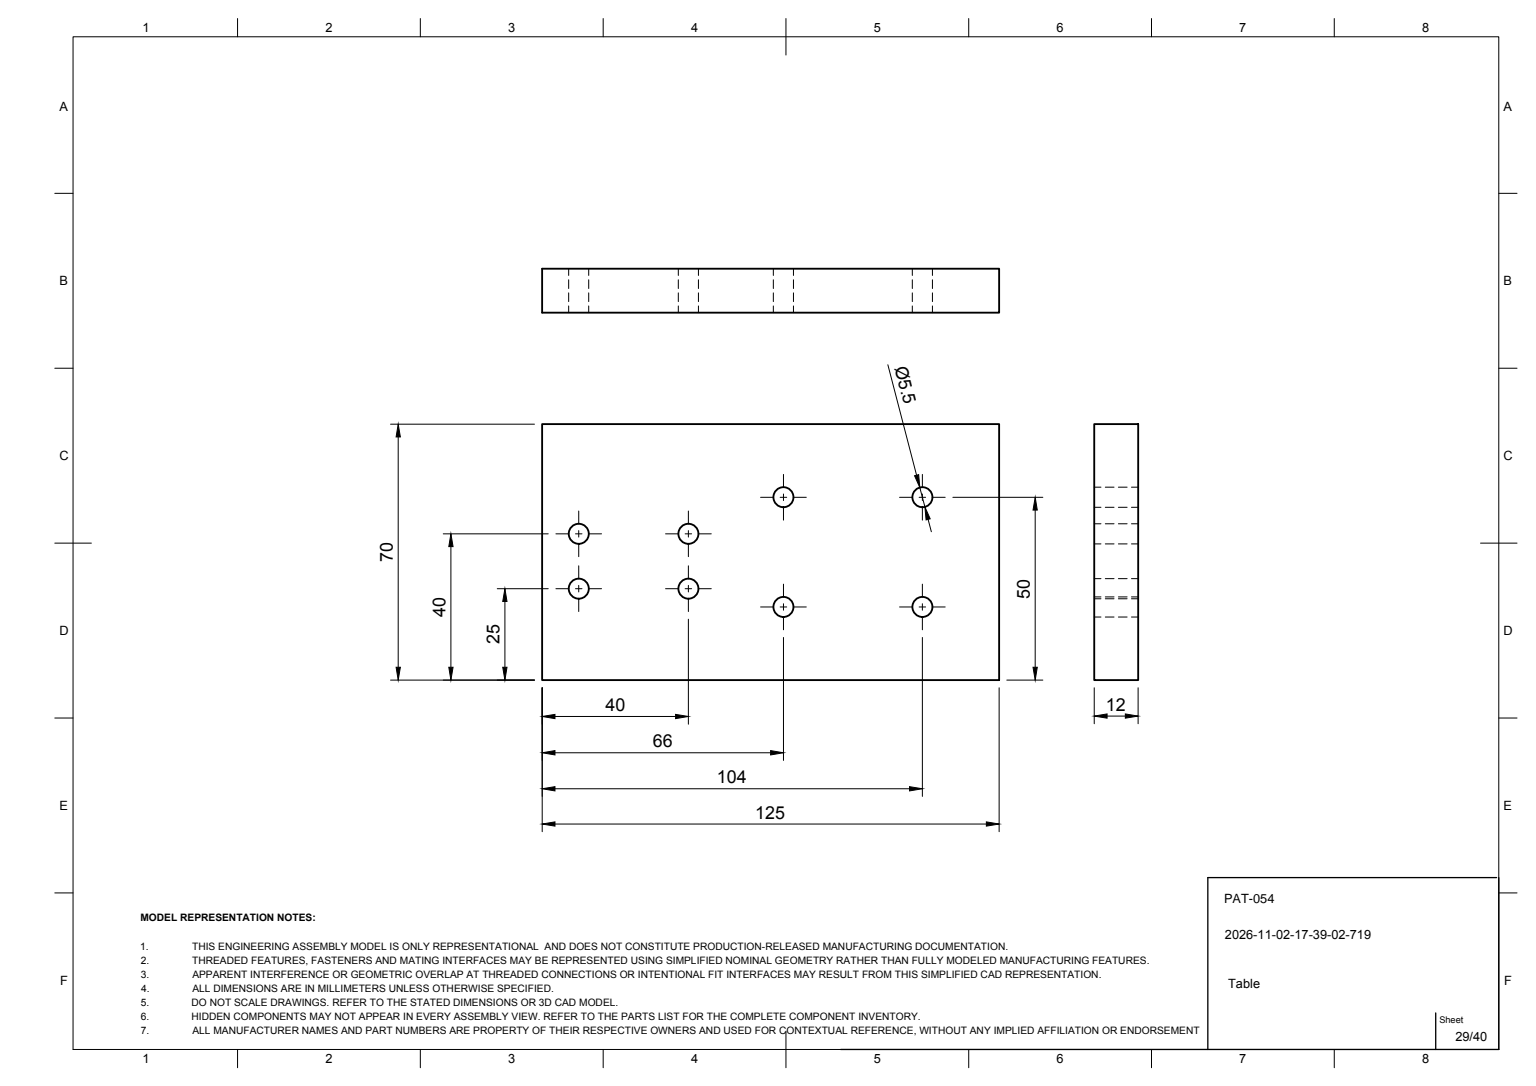
ISO-10303-21;
HEADER;
/* Generated by software containing ST-Developer
 * from STEP Tools, Inc. (www.steptools.com) 
 */

FILE_DESCRIPTION(
/* description */ ('PAT-054'),
/* implementation_level */ '2;1');

FILE_NAME(
/* name */ 'Table.step',
/* time_stamp */ '2026-10-29T16:38:13-07:00',
/* author */ (''),
/* organization */ (''),
/* preprocessor_version */ 'ST-DEVELOPER v20.2',
/* originating_system */ 'Autodesk Translation Framework v15.17.0.0',
/* authorisation */ '');

FILE_SCHEMA (('AUTOMOTIVE_DESIGN { 1 0 10303 214 3 1 1 }'));
ENDSEC;

DATA;
#10=MECHANICAL_DESIGN_GEOMETRIC_PRESENTATION_REPRESENTATION('',(#938),#33981);
#835=SHAPE_REPRESENTATION_RELATIONSHIP('SRR','None',#34211,#879);
#879=ADVANCED_BREP_SHAPE_REPRESENTATION('',(#996),#33959);
#938=STYLED_ITEM('',(#34531),#996);
#996=MANIFOLD_SOLID_BREP('Body1',#13050);
#1160=FACE_BOUND('',#2799,.T.);
#1161=FACE_BOUND('',#2800,.T.);
#1162=FACE_BOUND('',#2801,.T.);
#1163=FACE_BOUND('',#2802,.T.);
#1164=FACE_BOUND('',#2803,.T.);
#1165=FACE_BOUND('',#2804,.T.);
#1166=FACE_BOUND('',#2805,.T.);
#1167=FACE_BOUND('',#2806,.T.);
#1168=FACE_BOUND('',#2808,.T.);
#1169=FACE_BOUND('',#2809,.T.);
#1170=FACE_BOUND('',#2810,.T.);
#1171=FACE_BOUND('',#2811,.T.);
#1172=FACE_BOUND('',#2812,.T.);
#1173=FACE_BOUND('',#2813,.T.);
#1174=FACE_BOUND('',#2814,.T.);
#1175=FACE_BOUND('',#2815,.T.);
#1418=PLANE('',#14280);
#1419=PLANE('',#14281);
#1420=PLANE('',#14282);
#1421=PLANE('',#14283);
#1422=PLANE('',#14284);
#1423=PLANE('',#14285);
#1915=FACE_OUTER_BOUND('',#2786,.T.);
#1916=FACE_OUTER_BOUND('',#2787,.T.);
#1917=FACE_OUTER_BOUND('',#2788,.T.);
#1918=FACE_OUTER_BOUND('',#2789,.T.);
#1919=FACE_OUTER_BOUND('',#2790,.T.);
#1920=FACE_OUTER_BOUND('',#2791,.T.);
#1921=FACE_OUTER_BOUND('',#2792,.T.);
#1922=FACE_OUTER_BOUND('',#2793,.T.);
#1923=FACE_OUTER_BOUND('',#2794,.T.);
#1924=FACE_OUTER_BOUND('',#2795,.T.);
#1925=FACE_OUTER_BOUND('',#2796,.T.);
#1926=FACE_OUTER_BOUND('',#2797,.T.);
#1927=FACE_OUTER_BOUND('',#2798,.T.);
#1928=FACE_OUTER_BOUND('',#2807,.T.);
#2786=EDGE_LOOP('',(#10085,#10086,#10087,#10088));
#2787=EDGE_LOOP('',(#10089,#10090,#10091,#10092));
#2788=EDGE_LOOP('',(#10093,#10094,#10095,#10096));
#2789=EDGE_LOOP('',(#10097,#10098,#10099,#10100));
#2790=EDGE_LOOP('',(#10101,#10102,#10103,#10104));
#2791=EDGE_LOOP('',(#10105,#10106,#10107,#10108));
#2792=EDGE_LOOP('',(#10109,#10110,#10111,#10112));
#2793=EDGE_LOOP('',(#10113,#10114,#10115,#10116));
#2794=EDGE_LOOP('',(#10117,#10118,#10119,#10120));
#2795=EDGE_LOOP('',(#10121,#10122,#10123,#10124));
#2796=EDGE_LOOP('',(#10125,#10126,#10127,#10128));
#2797=EDGE_LOOP('',(#10129,#10130,#10131,#10132));
#2798=EDGE_LOOP('',(#10133,#10134,#10135,#10136));
#2799=EDGE_LOOP('',(#10137));
#2800=EDGE_LOOP('',(#10138));
#2801=EDGE_LOOP('',(#10139));
#2802=EDGE_LOOP('',(#10140));
#2803=EDGE_LOOP('',(#10141));
#2804=EDGE_LOOP('',(#10142));
#2805=EDGE_LOOP('',(#10143));
#2806=EDGE_LOOP('',(#10144));
#2807=EDGE_LOOP('',(#10145,#10146,#10147,#10148));
#2808=EDGE_LOOP('',(#10149));
#2809=EDGE_LOOP('',(#10150));
#2810=EDGE_LOOP('',(#10151));
#2811=EDGE_LOOP('',(#10152));
#2812=EDGE_LOOP('',(#10153));
#2813=EDGE_LOOP('',(#10154));
#2814=EDGE_LOOP('',(#10155));
#2815=EDGE_LOOP('',(#10156));
#3686=LINE('',#20848,#4620);
#3687=LINE('',#20854,#4621);
#3688=LINE('',#20860,#4622);
#3689=LINE('',#20866,#4623);
#3690=LINE('',#20872,#4624);
#3691=LINE('',#20878,#4625);
#3692=LINE('',#20884,#4626);
#3693=LINE('',#20890,#4627);
#3694=LINE('',#20895,#4628);
#3695=LINE('',#20897,#4629);
#3696=LINE('',#20899,#4630);
#3697=LINE('',#20900,#4631);
#3698=LINE('',#20903,#4632);
#3699=LINE('',#20905,#4633);
#3700=LINE('',#20906,#4634);
#3701=LINE('',#20909,#4635);
#3702=LINE('',#20911,#4636);
#3703=LINE('',#20912,#4637);
#3704=LINE('',#20914,#4638);
#3705=LINE('',#20915,#4639);
#4620=VECTOR('',#16737,0.275);
#4621=VECTOR('',#16744,0.275);
#4622=VECTOR('',#16751,0.275);
#4623=VECTOR('',#16758,0.275);
#4624=VECTOR('',#16765,0.275);
#4625=VECTOR('',#16772,0.275);
#4626=VECTOR('',#16779,0.275);
#4627=VECTOR('',#16786,0.275);
#4628=VECTOR('',#16791,1.);
#4629=VECTOR('',#16792,1.);
#4630=VECTOR('',#16793,1.);
#4631=VECTOR('',#16794,1.);
#4632=VECTOR('',#16797,1.);
#4633=VECTOR('',#16798,1.);
#4634=VECTOR('',#16799,1.);
#4635=VECTOR('',#16802,1.);
#4636=VECTOR('',#16803,1.);
#4637=VECTOR('',#16804,1.);
#4638=VECTOR('',#16807,1.);
#4639=VECTOR('',#16808,1.);
#5420=CIRCLE('',#14257,0.275);
#5421=CIRCLE('',#14258,0.275);
#5422=CIRCLE('',#14260,0.275);
#5423=CIRCLE('',#14261,0.275);
#5424=CIRCLE('',#14263,0.275);
#5425=CIRCLE('',#14264,0.275);
#5426=CIRCLE('',#14266,0.275);
#5427=CIRCLE('',#14267,0.275);
#5428=CIRCLE('',#14269,0.275);
#5429=CIRCLE('',#14270,0.275);
#5430=CIRCLE('',#14272,0.275);
#5431=CIRCLE('',#14273,0.275);
#5432=CIRCLE('',#14275,0.275);
#5433=CIRCLE('',#14276,0.275);
#5434=CIRCLE('',#14278,0.275);
#5435=CIRCLE('',#14279,0.275);
#6118=VERTEX_POINT('',#20845);
#6119=VERTEX_POINT('',#20847);
#6120=VERTEX_POINT('',#20851);
#6121=VERTEX_POINT('',#20853);
#6122=VERTEX_POINT('',#20857);
#6123=VERTEX_POINT('',#20859);
#6124=VERTEX_POINT('',#20863);
#6125=VERTEX_POINT('',#20865);
#6126=VERTEX_POINT('',#20869);
#6127=VERTEX_POINT('',#20871);
#6128=VERTEX_POINT('',#20875);
#6129=VERTEX_POINT('',#20877);
#6130=VERTEX_POINT('',#20881);
#6131=VERTEX_POINT('',#20883);
#6132=VERTEX_POINT('',#20887);
#6133=VERTEX_POINT('',#20889);
#6134=VERTEX_POINT('',#20893);
#6135=VERTEX_POINT('',#20894);
#6136=VERTEX_POINT('',#20896);
#6137=VERTEX_POINT('',#20898);
#6138=VERTEX_POINT('',#20902);
#6139=VERTEX_POINT('',#20904);
#6140=VERTEX_POINT('',#20908);
#6141=VERTEX_POINT('',#20910);
#7542=EDGE_CURVE('',#6118,#6118,#5420,.T.);
#7543=EDGE_CURVE('',#6118,#6119,#3686,.T.);
#7544=EDGE_CURVE('',#6119,#6119,#5421,.T.);
#7545=EDGE_CURVE('',#6120,#6120,#5422,.T.);
#7546=EDGE_CURVE('',#6120,#6121,#3687,.T.);
#7547=EDGE_CURVE('',#6121,#6121,#5423,.T.);
#7548=EDGE_CURVE('',#6122,#6122,#5424,.T.);
#7549=EDGE_CURVE('',#6122,#6123,#3688,.T.);
#7550=EDGE_CURVE('',#6123,#6123,#5425,.T.);
#7551=EDGE_CURVE('',#6124,#6124,#5426,.T.);
#7552=EDGE_CURVE('',#6124,#6125,#3689,.T.);
#7553=EDGE_CURVE('',#6125,#6125,#5427,.T.);
#7554=EDGE_CURVE('',#6126,#6126,#5428,.T.);
#7555=EDGE_CURVE('',#6126,#6127,#3690,.T.);
#7556=EDGE_CURVE('',#6127,#6127,#5429,.T.);
#7557=EDGE_CURVE('',#6128,#6128,#5430,.T.);
#7558=EDGE_CURVE('',#6128,#6129,#3691,.T.);
#7559=EDGE_CURVE('',#6129,#6129,#5431,.T.);
#7560=EDGE_CURVE('',#6130,#6130,#5432,.T.);
#7561=EDGE_CURVE('',#6130,#6131,#3692,.T.);
#7562=EDGE_CURVE('',#6131,#6131,#5433,.T.);
#7563=EDGE_CURVE('',#6132,#6132,#5434,.T.);
#7564=EDGE_CURVE('',#6132,#6133,#3693,.T.);
#7565=EDGE_CURVE('',#6133,#6133,#5435,.T.);
#7566=EDGE_CURVE('',#6134,#6135,#3694,.T.);
#7567=EDGE_CURVE('',#6135,#6136,#3695,.T.);
#7568=EDGE_CURVE('',#6137,#6136,#3696,.T.);
#7569=EDGE_CURVE('',#6134,#6137,#3697,.T.);
#7570=EDGE_CURVE('',#6138,#6134,#3698,.T.);
#7571=EDGE_CURVE('',#6139,#6137,#3699,.T.);
#7572=EDGE_CURVE('',#6138,#6139,#3700,.T.);
#7573=EDGE_CURVE('',#6140,#6138,#3701,.T.);
#7574=EDGE_CURVE('',#6141,#6139,#3702,.T.);
#7575=EDGE_CURVE('',#6140,#6141,#3703,.T.);
#7576=EDGE_CURVE('',#6135,#6140,#3704,.T.);
#7577=EDGE_CURVE('',#6136,#6141,#3705,.T.);
#10085=ORIENTED_EDGE('',*,*,#7542,.F.);
#10086=ORIENTED_EDGE('',*,*,#7543,.T.);
#10087=ORIENTED_EDGE('',*,*,#7544,.F.);
#10088=ORIENTED_EDGE('',*,*,#7543,.F.);
#10089=ORIENTED_EDGE('',*,*,#7545,.F.);
#10090=ORIENTED_EDGE('',*,*,#7546,.T.);
#10091=ORIENTED_EDGE('',*,*,#7547,.F.);
#10092=ORIENTED_EDGE('',*,*,#7546,.F.);
#10093=ORIENTED_EDGE('',*,*,#7548,.F.);
#10094=ORIENTED_EDGE('',*,*,#7549,.T.);
#10095=ORIENTED_EDGE('',*,*,#7550,.F.);
#10096=ORIENTED_EDGE('',*,*,#7549,.F.);
#10097=ORIENTED_EDGE('',*,*,#7551,.F.);
#10098=ORIENTED_EDGE('',*,*,#7552,.T.);
#10099=ORIENTED_EDGE('',*,*,#7553,.F.);
#10100=ORIENTED_EDGE('',*,*,#7552,.F.);
#10101=ORIENTED_EDGE('',*,*,#7554,.F.);
#10102=ORIENTED_EDGE('',*,*,#7555,.T.);
#10103=ORIENTED_EDGE('',*,*,#7556,.F.);
#10104=ORIENTED_EDGE('',*,*,#7555,.F.);
#10105=ORIENTED_EDGE('',*,*,#7557,.F.);
#10106=ORIENTED_EDGE('',*,*,#7558,.T.);
#10107=ORIENTED_EDGE('',*,*,#7559,.F.);
#10108=ORIENTED_EDGE('',*,*,#7558,.F.);
#10109=ORIENTED_EDGE('',*,*,#7560,.F.);
#10110=ORIENTED_EDGE('',*,*,#7561,.T.);
#10111=ORIENTED_EDGE('',*,*,#7562,.F.);
#10112=ORIENTED_EDGE('',*,*,#7561,.F.);
#10113=ORIENTED_EDGE('',*,*,#7563,.F.);
#10114=ORIENTED_EDGE('',*,*,#7564,.T.);
#10115=ORIENTED_EDGE('',*,*,#7565,.F.);
#10116=ORIENTED_EDGE('',*,*,#7564,.F.);
#10117=ORIENTED_EDGE('',*,*,#7566,.T.);
#10118=ORIENTED_EDGE('',*,*,#7567,.T.);
#10119=ORIENTED_EDGE('',*,*,#7568,.F.);
#10120=ORIENTED_EDGE('',*,*,#7569,.F.);
#10121=ORIENTED_EDGE('',*,*,#7570,.T.);
#10122=ORIENTED_EDGE('',*,*,#7569,.T.);
#10123=ORIENTED_EDGE('',*,*,#7571,.F.);
#10124=ORIENTED_EDGE('',*,*,#7572,.F.);
#10125=ORIENTED_EDGE('',*,*,#7573,.T.);
#10126=ORIENTED_EDGE('',*,*,#7572,.T.);
#10127=ORIENTED_EDGE('',*,*,#7574,.F.);
#10128=ORIENTED_EDGE('',*,*,#7575,.F.);
#10129=ORIENTED_EDGE('',*,*,#7576,.T.);
#10130=ORIENTED_EDGE('',*,*,#7575,.T.);
#10131=ORIENTED_EDGE('',*,*,#7577,.F.);
#10132=ORIENTED_EDGE('',*,*,#7567,.F.);
#10133=ORIENTED_EDGE('',*,*,#7577,.T.);
#10134=ORIENTED_EDGE('',*,*,#7574,.T.);
#10135=ORIENTED_EDGE('',*,*,#7571,.T.);
#10136=ORIENTED_EDGE('',*,*,#7568,.T.);
#10137=ORIENTED_EDGE('',*,*,#7565,.T.);
#10138=ORIENTED_EDGE('',*,*,#7562,.T.);
#10139=ORIENTED_EDGE('',*,*,#7559,.T.);
#10140=ORIENTED_EDGE('',*,*,#7556,.T.);
#10141=ORIENTED_EDGE('',*,*,#7553,.T.);
#10142=ORIENTED_EDGE('',*,*,#7550,.T.);
#10143=ORIENTED_EDGE('',*,*,#7547,.T.);
#10144=ORIENTED_EDGE('',*,*,#7544,.T.);
#10145=ORIENTED_EDGE('',*,*,#7576,.F.);
#10146=ORIENTED_EDGE('',*,*,#7566,.F.);
#10147=ORIENTED_EDGE('',*,*,#7570,.F.);
#10148=ORIENTED_EDGE('',*,*,#7573,.F.);
#10149=ORIENTED_EDGE('',*,*,#7563,.T.);
#10150=ORIENTED_EDGE('',*,*,#7560,.T.);
#10151=ORIENTED_EDGE('',*,*,#7557,.T.);
#10152=ORIENTED_EDGE('',*,*,#7554,.T.);
#10153=ORIENTED_EDGE('',*,*,#7551,.T.);
#10154=ORIENTED_EDGE('',*,*,#7548,.T.);
#10155=ORIENTED_EDGE('',*,*,#7545,.T.);
#10156=ORIENTED_EDGE('',*,*,#7542,.T.);
#12083=CYLINDRICAL_SURFACE('',#14256,0.275);
#12084=CYLINDRICAL_SURFACE('',#14259,0.275);
#12085=CYLINDRICAL_SURFACE('',#14262,0.275);
#12086=CYLINDRICAL_SURFACE('',#14265,0.275);
#12087=CYLINDRICAL_SURFACE('',#14268,0.275);
#12088=CYLINDRICAL_SURFACE('',#14271,0.275);
#12089=CYLINDRICAL_SURFACE('',#14274,0.275);
#12090=CYLINDRICAL_SURFACE('',#14277,0.275);
#12627=ADVANCED_FACE('',(#1915),#12083,.F.);
#12628=ADVANCED_FACE('',(#1916),#12084,.F.);
#12629=ADVANCED_FACE('',(#1917),#12085,.F.);
#12630=ADVANCED_FACE('',(#1918),#12086,.F.);
#12631=ADVANCED_FACE('',(#1919),#12087,.F.);
#12632=ADVANCED_FACE('',(#1920),#12088,.F.);
#12633=ADVANCED_FACE('',(#1921),#12089,.F.);
#12634=ADVANCED_FACE('',(#1922),#12090,.F.);
#12635=ADVANCED_FACE('',(#1923),#1418,.T.);
#12636=ADVANCED_FACE('',(#1924),#1419,.T.);
#12637=ADVANCED_FACE('',(#1925),#1420,.T.);
#12638=ADVANCED_FACE('',(#1926),#1421,.T.);
#12639=ADVANCED_FACE('',(#1927,#1160,#1161,#1162,#1163,#1164,#1165,#1166,
#1167),#1422,.T.);
#12640=ADVANCED_FACE('',(#1928,#1168,#1169,#1170,#1171,#1172,#1173,#1174,
#1175),#1423,.F.);
#13050=CLOSED_SHELL('',(#12627,#12628,#12629,#12630,#12631,#12632,#12633,
#12634,#12635,#12636,#12637,#12638,#12639,#12640));
#14255=AXIS2_PLACEMENT_3D('',#20843,#16731,#16732);
#14256=AXIS2_PLACEMENT_3D('',#20844,#16733,#16734);
#14257=AXIS2_PLACEMENT_3D('',#20846,#16735,#16736);
#14258=AXIS2_PLACEMENT_3D('',#20849,#16738,#16739);
#14259=AXIS2_PLACEMENT_3D('',#20850,#16740,#16741);
#14260=AXIS2_PLACEMENT_3D('',#20852,#16742,#16743);
#14261=AXIS2_PLACEMENT_3D('',#20855,#16745,#16746);
#14262=AXIS2_PLACEMENT_3D('',#20856,#16747,#16748);
#14263=AXIS2_PLACEMENT_3D('',#20858,#16749,#16750);
#14264=AXIS2_PLACEMENT_3D('',#20861,#16752,#16753);
#14265=AXIS2_PLACEMENT_3D('',#20862,#16754,#16755);
#14266=AXIS2_PLACEMENT_3D('',#20864,#16756,#16757);
#14267=AXIS2_PLACEMENT_3D('',#20867,#16759,#16760);
#14268=AXIS2_PLACEMENT_3D('',#20868,#16761,#16762);
#14269=AXIS2_PLACEMENT_3D('',#20870,#16763,#16764);
#14270=AXIS2_PLACEMENT_3D('',#20873,#16766,#16767);
#14271=AXIS2_PLACEMENT_3D('',#20874,#16768,#16769);
#14272=AXIS2_PLACEMENT_3D('',#20876,#16770,#16771);
#14273=AXIS2_PLACEMENT_3D('',#20879,#16773,#16774);
#14274=AXIS2_PLACEMENT_3D('',#20880,#16775,#16776);
#14275=AXIS2_PLACEMENT_3D('',#20882,#16777,#16778);
#14276=AXIS2_PLACEMENT_3D('',#20885,#16780,#16781);
#14277=AXIS2_PLACEMENT_3D('',#20886,#16782,#16783);
#14278=AXIS2_PLACEMENT_3D('',#20888,#16784,#16785);
#14279=AXIS2_PLACEMENT_3D('',#20891,#16787,#16788);
#14280=AXIS2_PLACEMENT_3D('',#20892,#16789,#16790);
#14281=AXIS2_PLACEMENT_3D('',#20901,#16795,#16796);
#14282=AXIS2_PLACEMENT_3D('',#20907,#16800,#16801);
#14283=AXIS2_PLACEMENT_3D('',#20913,#16805,#16806);
#14284=AXIS2_PLACEMENT_3D('',#20916,#16809,#16810);
#14285=AXIS2_PLACEMENT_3D('',#20917,#16811,#16812);
#16731=DIRECTION('axis',(0.,0.,1.));
#16732=DIRECTION('refdir',(1.,0.,0.));
#16733=DIRECTION('center_axis',(0.,0.,1.));
#16734=DIRECTION('ref_axis',(1.,0.,0.));
#16735=DIRECTION('center_axis',(0.,0.,1.));
#16736=DIRECTION('ref_axis',(1.,0.,0.));
#16737=DIRECTION('',(0.,0.,1.));
#16738=DIRECTION('center_axis',(0.,0.,-1.));
#16739=DIRECTION('ref_axis',(1.,0.,0.));
#16740=DIRECTION('center_axis',(0.,0.,1.));
#16741=DIRECTION('ref_axis',(1.,0.,0.));
#16742=DIRECTION('center_axis',(0.,0.,1.));
#16743=DIRECTION('ref_axis',(1.,0.,0.));
#16744=DIRECTION('',(0.,0.,1.));
#16745=DIRECTION('center_axis',(0.,0.,-1.));
#16746=DIRECTION('ref_axis',(1.,0.,0.));
#16747=DIRECTION('center_axis',(0.,0.,1.));
#16748=DIRECTION('ref_axis',(1.,0.,0.));
#16749=DIRECTION('center_axis',(0.,0.,1.));
#16750=DIRECTION('ref_axis',(1.,0.,0.));
#16751=DIRECTION('',(0.,0.,1.));
#16752=DIRECTION('center_axis',(0.,0.,-1.));
#16753=DIRECTION('ref_axis',(1.,0.,0.));
#16754=DIRECTION('center_axis',(0.,0.,1.));
#16755=DIRECTION('ref_axis',(1.,0.,0.));
#16756=DIRECTION('center_axis',(0.,0.,1.));
#16757=DIRECTION('ref_axis',(1.,0.,0.));
#16758=DIRECTION('',(0.,0.,1.));
#16759=DIRECTION('center_axis',(0.,0.,-1.));
#16760=DIRECTION('ref_axis',(1.,0.,0.));
#16761=DIRECTION('center_axis',(0.,0.,1.));
#16762=DIRECTION('ref_axis',(1.,0.,0.));
#16763=DIRECTION('center_axis',(0.,0.,1.));
#16764=DIRECTION('ref_axis',(1.,0.,0.));
#16765=DIRECTION('',(0.,0.,1.));
#16766=DIRECTION('center_axis',(0.,0.,-1.));
#16767=DIRECTION('ref_axis',(1.,0.,0.));
#16768=DIRECTION('center_axis',(0.,0.,1.));
#16769=DIRECTION('ref_axis',(1.,0.,0.));
#16770=DIRECTION('center_axis',(0.,0.,1.));
#16771=DIRECTION('ref_axis',(1.,0.,0.));
#16772=DIRECTION('',(0.,0.,1.));
#16773=DIRECTION('center_axis',(0.,0.,-1.));
#16774=DIRECTION('ref_axis',(1.,0.,0.));
#16775=DIRECTION('center_axis',(0.,0.,1.));
#16776=DIRECTION('ref_axis',(1.,0.,0.));
#16777=DIRECTION('center_axis',(0.,0.,1.));
#16778=DIRECTION('ref_axis',(1.,0.,0.));
#16779=DIRECTION('',(0.,0.,1.));
#16780=DIRECTION('center_axis',(0.,0.,-1.));
#16781=DIRECTION('ref_axis',(1.,0.,0.));
#16782=DIRECTION('center_axis',(0.,0.,1.));
#16783=DIRECTION('ref_axis',(1.,0.,0.));
#16784=DIRECTION('center_axis',(0.,0.,1.));
#16785=DIRECTION('ref_axis',(1.,0.,0.));
#16786=DIRECTION('',(0.,0.,1.));
#16787=DIRECTION('center_axis',(0.,0.,-1.));
#16788=DIRECTION('ref_axis',(1.,0.,0.));
#16789=DIRECTION('center_axis',(0.,1.,0.));
#16790=DIRECTION('ref_axis',(-1.,0.,0.));
#16791=DIRECTION('',(-1.,0.,0.));
#16792=DIRECTION('',(0.,0.,1.));
#16793=DIRECTION('',(-1.,0.,0.));
#16794=DIRECTION('',(0.,0.,1.));
#16795=DIRECTION('center_axis',(1.,0.,0.));
#16796=DIRECTION('ref_axis',(0.,1.,0.));
#16797=DIRECTION('',(0.,1.,0.));
#16798=DIRECTION('',(0.,1.,0.));
#16799=DIRECTION('',(0.,0.,1.));
#16800=DIRECTION('center_axis',(0.,-1.,0.));
#16801=DIRECTION('ref_axis',(1.,0.,0.));
#16802=DIRECTION('',(1.,0.,0.));
#16803=DIRECTION('',(1.,0.,0.));
#16804=DIRECTION('',(0.,0.,1.));
#16805=DIRECTION('center_axis',(-1.,0.,0.));
#16806=DIRECTION('ref_axis',(0.,-1.,0.));
#16807=DIRECTION('',(0.,-1.,0.));
#16808=DIRECTION('',(0.,-1.,0.));
#16809=DIRECTION('center_axis',(0.,0.,1.));
#16810=DIRECTION('ref_axis',(1.,0.,0.));
#16811=DIRECTION('center_axis',(0.,0.,1.));
#16812=DIRECTION('ref_axis',(1.,0.,0.));
#20843=CARTESIAN_POINT('',(0.,0.,0.));
#20844=CARTESIAN_POINT('Origin',(14.,-1.5,5.9));
#20845=CARTESIAN_POINT('',(13.725,-1.5,6.));
#20846=CARTESIAN_POINT('Origin',(14.,-1.5,6.));
#20847=CARTESIAN_POINT('',(13.725,-1.5,7.2));
#20848=CARTESIAN_POINT('',(13.725,-1.5,5.9));
#20849=CARTESIAN_POINT('Origin',(14.,-1.5,7.2));
#20850=CARTESIAN_POINT('Origin',(12.5,1.5,5.9));
#20851=CARTESIAN_POINT('',(12.225,1.5,6.));
#20852=CARTESIAN_POINT('Origin',(12.5,1.5,6.));
#20853=CARTESIAN_POINT('',(12.225,1.5,7.2));
#20854=CARTESIAN_POINT('',(12.225,1.5,5.9));
#20855=CARTESIAN_POINT('Origin',(12.5,1.5,7.2));
#20856=CARTESIAN_POINT('Origin',(12.5,-1.5,5.9));
#20857=CARTESIAN_POINT('',(12.225,-1.5,6.));
#20858=CARTESIAN_POINT('Origin',(12.5,-1.5,6.));
#20859=CARTESIAN_POINT('',(12.225,-1.5,7.2));
#20860=CARTESIAN_POINT('',(12.225,-1.5,5.9));
#20861=CARTESIAN_POINT('Origin',(12.5,-1.5,7.2));
#20862=CARTESIAN_POINT('Origin',(14.,1.5,5.9));
#20863=CARTESIAN_POINT('',(13.725,1.5,6.));
#20864=CARTESIAN_POINT('Origin',(14.,1.5,6.));
#20865=CARTESIAN_POINT('',(13.725,1.5,7.2));
#20866=CARTESIAN_POINT('',(13.725,1.5,5.9));
#20867=CARTESIAN_POINT('Origin',(14.,1.5,7.2));
#20868=CARTESIAN_POINT('Origin',(15.,-7.9,5.1));
#20869=CARTESIAN_POINT('',(14.725,-7.9,6.));
#20870=CARTESIAN_POINT('Origin',(15.,-7.9,6.));
#20871=CARTESIAN_POINT('',(14.725,-7.9,7.2));
#20872=CARTESIAN_POINT('',(14.725,-7.9,5.1));
#20873=CARTESIAN_POINT('Origin',(15.,-7.9,7.2));
#20874=CARTESIAN_POINT('Origin',(12.,-4.1,5.1));
#20875=CARTESIAN_POINT('',(11.725,-4.1,6.));
#20876=CARTESIAN_POINT('Origin',(12.,-4.1,6.));
#20877=CARTESIAN_POINT('',(11.725,-4.1,7.2));
#20878=CARTESIAN_POINT('',(11.725,-4.1,5.1));
#20879=CARTESIAN_POINT('Origin',(12.,-4.1,7.2));
#20880=CARTESIAN_POINT('Origin',(12.,-7.9,5.1));
#20881=CARTESIAN_POINT('',(11.725,-7.9,6.));
#20882=CARTESIAN_POINT('Origin',(12.,-7.9,6.));
#20883=CARTESIAN_POINT('',(11.725,-7.9,7.2));
#20884=CARTESIAN_POINT('',(11.725,-7.9,5.1));
#20885=CARTESIAN_POINT('Origin',(12.,-7.9,7.2));
#20886=CARTESIAN_POINT('Origin',(15.,-4.1,5.1));
#20887=CARTESIAN_POINT('',(14.725,-4.1,6.));
#20888=CARTESIAN_POINT('Origin',(15.,-4.1,6.));
#20889=CARTESIAN_POINT('',(14.725,-4.1,7.2));
#20890=CARTESIAN_POINT('',(14.725,-4.1,5.1));
#20891=CARTESIAN_POINT('Origin',(15.,-4.1,7.2));
#20892=CARTESIAN_POINT('Origin',(17.,2.5,6.));
#20893=CARTESIAN_POINT('',(17.,2.5,6.));
#20894=CARTESIAN_POINT('',(10.,2.5,6.));
#20895=CARTESIAN_POINT('',(17.,2.5,6.));
#20896=CARTESIAN_POINT('',(10.,2.5,7.2));
#20897=CARTESIAN_POINT('',(10.,2.5,6.));
#20898=CARTESIAN_POINT('',(17.,2.5,7.2));
#20899=CARTESIAN_POINT('',(17.,2.5,7.2));
#20900=CARTESIAN_POINT('',(17.,2.5,6.));
#20901=CARTESIAN_POINT('Origin',(17.,-10.,6.));
#20902=CARTESIAN_POINT('',(17.,-10.,6.));
#20903=CARTESIAN_POINT('',(17.,-10.,6.));
#20904=CARTESIAN_POINT('',(17.,-10.,7.2));
#20905=CARTESIAN_POINT('',(17.,-10.,7.2));
#20906=CARTESIAN_POINT('',(17.,-10.,6.));
#20907=CARTESIAN_POINT('Origin',(10.,-10.,6.));
#20908=CARTESIAN_POINT('',(10.,-10.,6.));
#20909=CARTESIAN_POINT('',(10.,-10.,6.));
#20910=CARTESIAN_POINT('',(10.,-10.,7.2));
#20911=CARTESIAN_POINT('',(10.,-10.,7.2));
#20912=CARTESIAN_POINT('',(10.,-10.,6.));
#20913=CARTESIAN_POINT('Origin',(10.,2.5,6.));
#20914=CARTESIAN_POINT('',(10.,2.5,6.));
#20915=CARTESIAN_POINT('',(10.,2.5,7.2));
#20916=CARTESIAN_POINT('Origin',(13.5,-3.75,7.2));
#20917=CARTESIAN_POINT('Origin',(13.5,-3.75,6.));
#33907=UNCERTAINTY_MEASURE_WITH_UNIT(LENGTH_MEASURE(0.001),#33982,
'DISTANCE_ACCURACY_VALUE',
'Maximum model space distance between geometric entities at asserted c
onnectivities');
#33929=UNCERTAINTY_MEASURE_WITH_UNIT(LENGTH_MEASURE(0.001),#33982,
'DISTANCE_ACCURACY_VALUE',
'Maximum model space distance between geometric entities at asserted c
onnectivities');
#33959=(
GEOMETRIC_REPRESENTATION_CONTEXT(3)
GLOBAL_UNCERTAINTY_ASSIGNED_CONTEXT((#33907))
GLOBAL_UNIT_ASSIGNED_CONTEXT((#33982,#33984,#33985))
REPRESENTATION_CONTEXT('','3D')
);
#33981=(
GEOMETRIC_REPRESENTATION_CONTEXT(3)
GLOBAL_UNCERTAINTY_ASSIGNED_CONTEXT((#33929))
GLOBAL_UNIT_ASSIGNED_CONTEXT((#33982,#33984,#33985))
REPRESENTATION_CONTEXT('','3D')
);
#33982=(
LENGTH_UNIT()
NAMED_UNIT(*)
SI_UNIT(.CENTI.,.METRE.)
);
#33984=(
NAMED_UNIT(*)
PLANE_ANGLE_UNIT()
SI_UNIT($,.RADIAN.)
);
#33985=(
NAMED_UNIT(*)
SI_UNIT($,.STERADIAN.)
SOLID_ANGLE_UNIT()
);
#34015=SHAPE_DEFINITION_REPRESENTATION(#34076,#34211);
#34076=PRODUCT_DEFINITION_SHAPE('',$,#34263);
#34211=SHAPE_REPRESENTATION('',(#14255),#33959);
#34233=PRODUCT_DEFINITION_CONTEXT('part definition',#34388,'design');
#34263=PRODUCT_DEFINITION('Table','Table',#34314,#34233);
#34314=PRODUCT_DEFINITION_FORMATION('',$,#34419);
#34388=APPLICATION_CONTEXT(
'Core Data for Automotive Mechanical Design Process');
#34389=PRODUCT_CONTEXT('part definition',#34388,'mechanical');
#34419=PRODUCT('Table','Table','Table',(#34389));
#34525=COLOUR_RGB('Off White',0.89,0.88,0.83);
#34526=FILL_AREA_STYLE_COLOUR('',#34525);
#34527=FILL_AREA_STYLE('',(#34526));
#34528=SURFACE_STYLE_FILL_AREA(#34527);
#34529=SURFACE_SIDE_STYLE('',(#34528));
#34530=SURFACE_STYLE_USAGE(.BOTH.,#34529);
#34531=PRESENTATION_STYLE_ASSIGNMENT((#34530));
ENDSEC;
END-ISO-10303-21;
